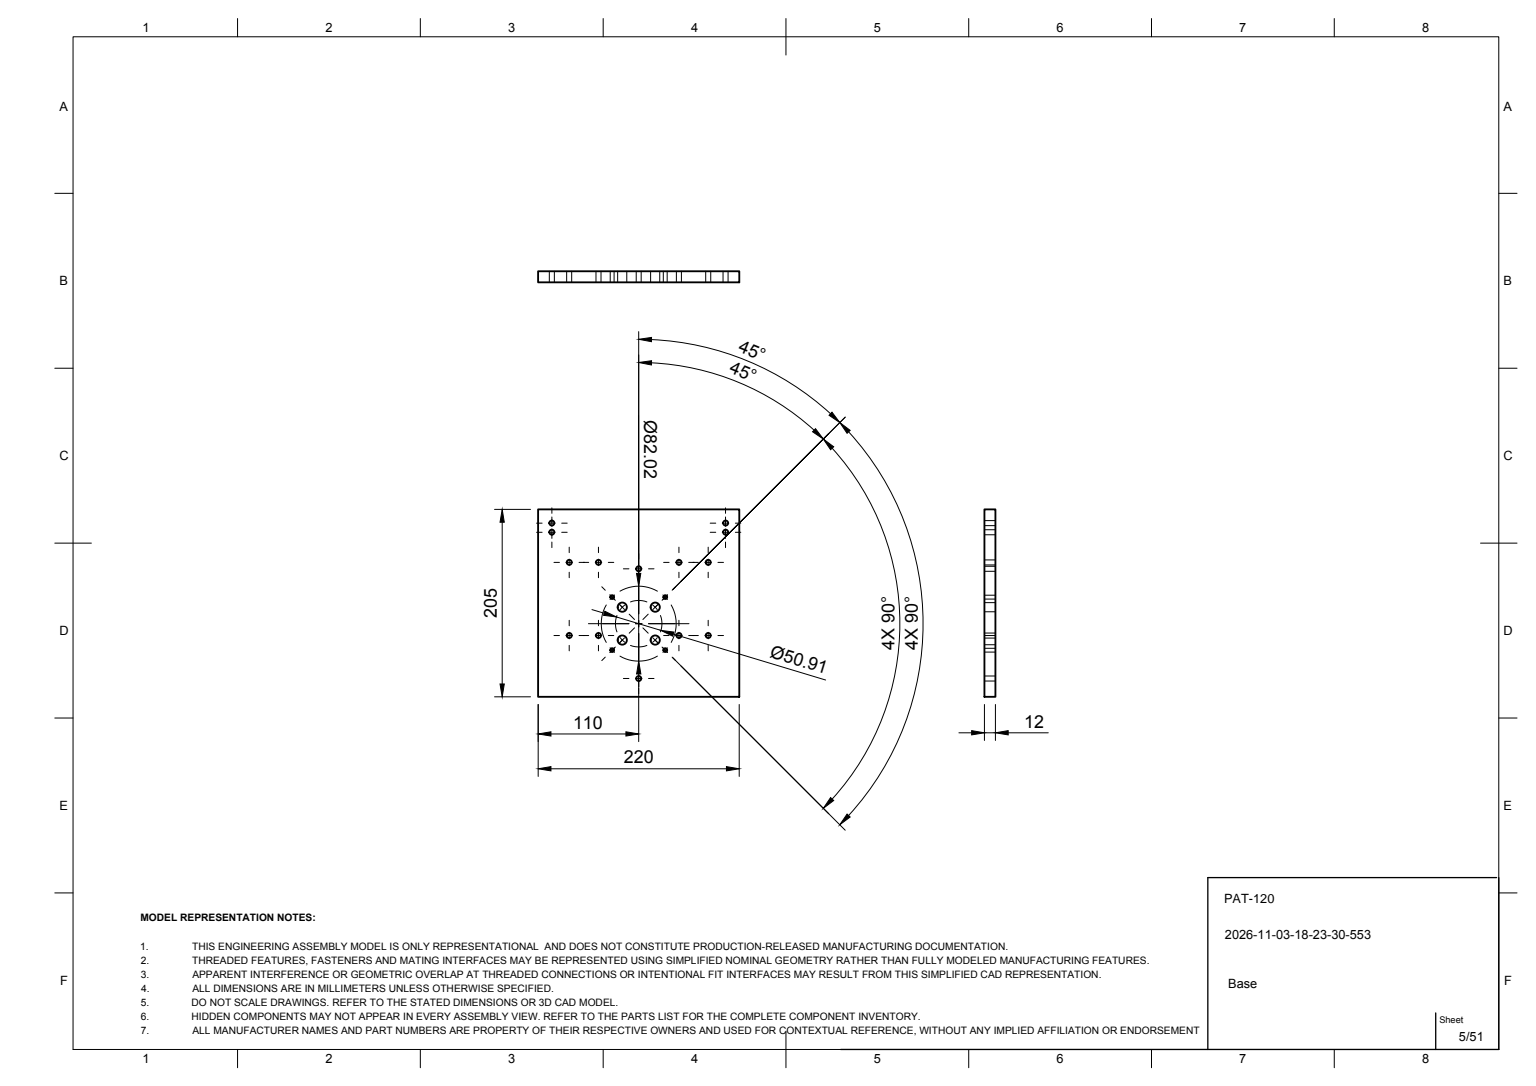
ISO-10303-21;
HEADER;
/* Generated by software containing ST-Developer
 * from STEP Tools, Inc. (www.steptools.com) 
 */

FILE_DESCRIPTION(
/* description */ ('Vibration shaker table dummy'),
/* implementation_level */ '2;1');

FILE_NAME(
/* name */ 'Base.step',
/* time_stamp */ '2026-10-27T10:55:14-07:00',
/* author */ (''),
/* organization */ (''),
/* preprocessor_version */ 'ST-DEVELOPER v20.2',
/* originating_system */ 'Autodesk Translation Framework v15.17.0.0',
/* authorisation */ '');

FILE_SCHEMA (('AUTOMOTIVE_DESIGN { 1 0 10303 214 3 1 1 }'));
ENDSEC;

DATA;
#10=MECHANICAL_DESIGN_GEOMETRIC_PRESENTATION_REPRESENTATION('',(#686),#22394);
#594=SHAPE_REPRESENTATION_RELATIONSHIP('SRR','None',#22640,#640);
#640=ADVANCED_BREP_SHAPE_REPRESENTATION('',(#732),#22346);
#686=STYLED_ITEM('',(#22940),#732);
#732=MANIFOLD_SOLID_BREP('Body1',#9204);
#775=FACE_BOUND('',#1866,.T.);
#776=FACE_BOUND('',#1867,.T.);
#777=FACE_BOUND('',#1868,.T.);
#778=FACE_BOUND('',#1869,.T.);
#779=FACE_BOUND('',#1870,.T.);
#780=FACE_BOUND('',#1871,.T.);
#781=FACE_BOUND('',#1872,.T.);
#782=FACE_BOUND('',#1873,.T.);
#783=FACE_BOUND('',#1874,.T.);
#784=FACE_BOUND('',#1875,.T.);
#785=FACE_BOUND('',#1876,.T.);
#786=FACE_BOUND('',#1877,.T.);
#787=FACE_BOUND('',#1878,.T.);
#788=FACE_BOUND('',#1879,.T.);
#789=FACE_BOUND('',#1880,.T.);
#790=FACE_BOUND('',#1881,.T.);
#791=FACE_BOUND('',#1882,.T.);
#792=FACE_BOUND('',#1883,.T.);
#793=FACE_BOUND('',#1884,.T.);
#794=FACE_BOUND('',#1885,.T.);
#795=FACE_BOUND('',#1886,.T.);
#796=FACE_BOUND('',#1887,.T.);
#797=FACE_BOUND('',#1889,.T.);
#798=FACE_BOUND('',#1890,.T.);
#799=FACE_BOUND('',#1891,.T.);
#800=FACE_BOUND('',#1892,.T.);
#801=FACE_BOUND('',#1893,.T.);
#802=FACE_BOUND('',#1894,.T.);
#803=FACE_BOUND('',#1895,.T.);
#804=FACE_BOUND('',#1896,.T.);
#805=FACE_BOUND('',#1897,.T.);
#806=FACE_BOUND('',#1898,.T.);
#807=FACE_BOUND('',#1899,.T.);
#808=FACE_BOUND('',#1900,.T.);
#809=FACE_BOUND('',#1901,.T.);
#810=FACE_BOUND('',#1902,.T.);
#811=FACE_BOUND('',#1903,.T.);
#812=FACE_BOUND('',#1904,.T.);
#813=FACE_BOUND('',#1905,.T.);
#814=FACE_BOUND('',#1906,.T.);
#815=FACE_BOUND('',#1907,.T.);
#816=FACE_BOUND('',#1908,.T.);
#817=FACE_BOUND('',#1909,.T.);
#818=FACE_BOUND('',#1910,.T.);
#1060=PLANE('',#9829);
#1061=PLANE('',#9830);
#1062=PLANE('',#9831);
#1063=PLANE('',#9832);
#1064=PLANE('',#9833);
#1065=PLANE('',#9834);
#1341=FACE_OUTER_BOUND('',#1839,.T.);
#1342=FACE_OUTER_BOUND('',#1840,.T.);
#1343=FACE_OUTER_BOUND('',#1841,.T.);
#1344=FACE_OUTER_BOUND('',#1842,.T.);
#1345=FACE_OUTER_BOUND('',#1843,.T.);
#1346=FACE_OUTER_BOUND('',#1844,.T.);
#1347=FACE_OUTER_BOUND('',#1845,.T.);
#1348=FACE_OUTER_BOUND('',#1846,.T.);
#1349=FACE_OUTER_BOUND('',#1847,.T.);
#1350=FACE_OUTER_BOUND('',#1848,.T.);
#1351=FACE_OUTER_BOUND('',#1849,.T.);
#1352=FACE_OUTER_BOUND('',#1850,.T.);
#1353=FACE_OUTER_BOUND('',#1851,.T.);
#1354=FACE_OUTER_BOUND('',#1852,.T.);
#1355=FACE_OUTER_BOUND('',#1853,.T.);
#1356=FACE_OUTER_BOUND('',#1854,.T.);
#1357=FACE_OUTER_BOUND('',#1855,.T.);
#1358=FACE_OUTER_BOUND('',#1856,.T.);
#1359=FACE_OUTER_BOUND('',#1857,.T.);
#1360=FACE_OUTER_BOUND('',#1858,.T.);
#1361=FACE_OUTER_BOUND('',#1859,.T.);
#1362=FACE_OUTER_BOUND('',#1860,.T.);
#1363=FACE_OUTER_BOUND('',#1861,.T.);
#1364=FACE_OUTER_BOUND('',#1862,.T.);
#1365=FACE_OUTER_BOUND('',#1863,.T.);
#1366=FACE_OUTER_BOUND('',#1864,.T.);
#1367=FACE_OUTER_BOUND('',#1865,.T.);
#1368=FACE_OUTER_BOUND('',#1888,.T.);
#1839=EDGE_LOOP('',(#6246,#6247,#6248,#6249));
#1840=EDGE_LOOP('',(#6250,#6251,#6252,#6253));
#1841=EDGE_LOOP('',(#6254,#6255,#6256,#6257));
#1842=EDGE_LOOP('',(#6258,#6259,#6260,#6261));
#1843=EDGE_LOOP('',(#6262,#6263,#6264,#6265));
#1844=EDGE_LOOP('',(#6266,#6267,#6268,#6269));
#1845=EDGE_LOOP('',(#6270,#6271,#6272,#6273));
#1846=EDGE_LOOP('',(#6274,#6275,#6276,#6277));
#1847=EDGE_LOOP('',(#6278,#6279,#6280,#6281));
#1848=EDGE_LOOP('',(#6282,#6283,#6284,#6285));
#1849=EDGE_LOOP('',(#6286,#6287,#6288,#6289));
#1850=EDGE_LOOP('',(#6290,#6291,#6292,#6293));
#1851=EDGE_LOOP('',(#6294,#6295,#6296,#6297));
#1852=EDGE_LOOP('',(#6298,#6299,#6300,#6301));
#1853=EDGE_LOOP('',(#6302,#6303,#6304,#6305));
#1854=EDGE_LOOP('',(#6306,#6307,#6308,#6309));
#1855=EDGE_LOOP('',(#6310,#6311,#6312,#6313));
#1856=EDGE_LOOP('',(#6314,#6315,#6316,#6317));
#1857=EDGE_LOOP('',(#6318,#6319,#6320,#6321));
#1858=EDGE_LOOP('',(#6322,#6323,#6324,#6325));
#1859=EDGE_LOOP('',(#6326,#6327,#6328,#6329));
#1860=EDGE_LOOP('',(#6330,#6331,#6332,#6333));
#1861=EDGE_LOOP('',(#6334,#6335,#6336,#6337));
#1862=EDGE_LOOP('',(#6338,#6339,#6340,#6341));
#1863=EDGE_LOOP('',(#6342,#6343,#6344,#6345));
#1864=EDGE_LOOP('',(#6346,#6347,#6348,#6349));
#1865=EDGE_LOOP('',(#6350,#6351,#6352,#6353));
#1866=EDGE_LOOP('',(#6354));
#1867=EDGE_LOOP('',(#6355));
#1868=EDGE_LOOP('',(#6356));
#1869=EDGE_LOOP('',(#6357));
#1870=EDGE_LOOP('',(#6358));
#1871=EDGE_LOOP('',(#6359));
#1872=EDGE_LOOP('',(#6360));
#1873=EDGE_LOOP('',(#6361));
#1874=EDGE_LOOP('',(#6362));
#1875=EDGE_LOOP('',(#6363));
#1876=EDGE_LOOP('',(#6364));
#1877=EDGE_LOOP('',(#6365));
#1878=EDGE_LOOP('',(#6366));
#1879=EDGE_LOOP('',(#6367));
#1880=EDGE_LOOP('',(#6368));
#1881=EDGE_LOOP('',(#6369));
#1882=EDGE_LOOP('',(#6370));
#1883=EDGE_LOOP('',(#6371));
#1884=EDGE_LOOP('',(#6372));
#1885=EDGE_LOOP('',(#6373));
#1886=EDGE_LOOP('',(#6374));
#1887=EDGE_LOOP('',(#6375));
#1888=EDGE_LOOP('',(#6376,#6377,#6378,#6379));
#1889=EDGE_LOOP('',(#6380));
#1890=EDGE_LOOP('',(#6381));
#1891=EDGE_LOOP('',(#6382));
#1892=EDGE_LOOP('',(#6383));
#1893=EDGE_LOOP('',(#6384));
#1894=EDGE_LOOP('',(#6385));
#1895=EDGE_LOOP('',(#6386));
#1896=EDGE_LOOP('',(#6387));
#1897=EDGE_LOOP('',(#6388));
#1898=EDGE_LOOP('',(#6389));
#1899=EDGE_LOOP('',(#6390));
#1900=EDGE_LOOP('',(#6391));
#1901=EDGE_LOOP('',(#6392));
#1902=EDGE_LOOP('',(#6393));
#1903=EDGE_LOOP('',(#6394));
#1904=EDGE_LOOP('',(#6395));
#1905=EDGE_LOOP('',(#6396));
#1906=EDGE_LOOP('',(#6397));
#1907=EDGE_LOOP('',(#6398));
#1908=EDGE_LOOP('',(#6399));
#1909=EDGE_LOOP('',(#6400));
#1910=EDGE_LOOP('',(#6401));
#2622=LINE('',#13956,#3241);
#2623=LINE('',#13962,#3242);
#2624=LINE('',#13968,#3243);
#2625=LINE('',#13974,#3244);
#2626=LINE('',#13980,#3245);
#2627=LINE('',#13986,#3246);
#2628=LINE('',#13992,#3247);
#2629=LINE('',#13998,#3248);
#2630=LINE('',#14004,#3249);
#2631=LINE('',#14010,#3250);
#2632=LINE('',#14016,#3251);
#2633=LINE('',#14022,#3252);
#2634=LINE('',#14028,#3253);
#2635=LINE('',#14034,#3254);
#2636=LINE('',#14040,#3255);
#2637=LINE('',#14046,#3256);
#2638=LINE('',#14052,#3257);
#2639=LINE('',#14058,#3258);
#2640=LINE('',#14064,#3259);
#2641=LINE('',#14070,#3260);
#2642=LINE('',#14076,#3261);
#2643=LINE('',#14082,#3262);
#2644=LINE('',#14087,#3263);
#2645=LINE('',#14089,#3264);
#2646=LINE('',#14091,#3265);
#2647=LINE('',#14092,#3266);
#2648=LINE('',#14095,#3267);
#2649=LINE('',#14097,#3268);
#2650=LINE('',#14098,#3269);
#2651=LINE('',#14101,#3270);
#2652=LINE('',#14103,#3271);
#2653=LINE('',#14104,#3272);
#2654=LINE('',#14106,#3273);
#2655=LINE('',#14107,#3274);
#3241=VECTOR('',#10960,0.275);
#3242=VECTOR('',#10967,0.275);
#3243=VECTOR('',#10974,0.5);
#3244=VECTOR('',#10981,0.5);
#3245=VECTOR('',#10988,0.5);
#3246=VECTOR('',#10995,0.5);
#3247=VECTOR('',#11002,0.21);
#3248=VECTOR('',#11009,0.21);
#3249=VECTOR('',#11016,0.21);
#3250=VECTOR('',#11023,0.21);
#3251=VECTOR('',#11030,0.275);
#3252=VECTOR('',#11037,0.275);
#3253=VECTOR('',#11044,0.275);
#3254=VECTOR('',#11051,0.275);
#3255=VECTOR('',#11058,0.275);
#3256=VECTOR('',#11065,0.275);
#3257=VECTOR('',#11072,0.275);
#3258=VECTOR('',#11079,0.275);
#3259=VECTOR('',#11086,0.275);
#3260=VECTOR('',#11093,0.275);
#3261=VECTOR('',#11100,0.275);
#3262=VECTOR('',#11107,0.275);
#3263=VECTOR('',#11112,1.);
#3264=VECTOR('',#11113,1.);
#3265=VECTOR('',#11114,1.);
#3266=VECTOR('',#11115,1.);
#3267=VECTOR('',#11118,1.);
#3268=VECTOR('',#11119,1.);
#3269=VECTOR('',#11120,1.);
#3270=VECTOR('',#11123,1.);
#3271=VECTOR('',#11124,1.);
#3272=VECTOR('',#11125,1.);
#3273=VECTOR('',#11128,1.);
#3274=VECTOR('',#11129,1.);
#3860=CIRCLE('',#9764,0.275);
#3861=CIRCLE('',#9765,0.275);
#3862=CIRCLE('',#9767,0.275);
#3863=CIRCLE('',#9768,0.275);
#3864=CIRCLE('',#9770,0.5);
#3865=CIRCLE('',#9771,0.5);
#3866=CIRCLE('',#9773,0.5);
#3867=CIRCLE('',#9774,0.5);
#3868=CIRCLE('',#9776,0.5);
#3869=CIRCLE('',#9777,0.5);
#3870=CIRCLE('',#9779,0.5);
#3871=CIRCLE('',#9780,0.5);
#3872=CIRCLE('',#9782,0.21);
#3873=CIRCLE('',#9783,0.21);
#3874=CIRCLE('',#9785,0.21);
#3875=CIRCLE('',#9786,0.21);
#3876=CIRCLE('',#9788,0.21);
#3877=CIRCLE('',#9789,0.21);
#3878=CIRCLE('',#9791,0.21);
#3879=CIRCLE('',#9792,0.21);
#3880=CIRCLE('',#9794,0.275);
#3881=CIRCLE('',#9795,0.275);
#3882=CIRCLE('',#9797,0.275);
#3883=CIRCLE('',#9798,0.275);
#3884=CIRCLE('',#9800,0.275);
#3885=CIRCLE('',#9801,0.275);
#3886=CIRCLE('',#9803,0.275);
#3887=CIRCLE('',#9804,0.275);
#3888=CIRCLE('',#9806,0.275);
#3889=CIRCLE('',#9807,0.275);
#3890=CIRCLE('',#9809,0.275);
#3891=CIRCLE('',#9810,0.275);
#3892=CIRCLE('',#9812,0.275);
#3893=CIRCLE('',#9813,0.275);
#3894=CIRCLE('',#9815,0.275);
#3895=CIRCLE('',#9816,0.275);
#3896=CIRCLE('',#9818,0.275);
#3897=CIRCLE('',#9819,0.275);
#3898=CIRCLE('',#9821,0.275);
#3899=CIRCLE('',#9822,0.275);
#3900=CIRCLE('',#9824,0.275);
#3901=CIRCLE('',#9825,0.275);
#3902=CIRCLE('',#9827,0.275);
#3903=CIRCLE('',#9828,0.275);
#4367=VERTEX_POINT('',#13953);
#4368=VERTEX_POINT('',#13955);
#4369=VERTEX_POINT('',#13959);
#4370=VERTEX_POINT('',#13961);
#4371=VERTEX_POINT('',#13965);
#4372=VERTEX_POINT('',#13967);
#4373=VERTEX_POINT('',#13971);
#4374=VERTEX_POINT('',#13973);
#4375=VERTEX_POINT('',#13977);
#4376=VERTEX_POINT('',#13979);
#4377=VERTEX_POINT('',#13983);
#4378=VERTEX_POINT('',#13985);
#4379=VERTEX_POINT('',#13989);
#4380=VERTEX_POINT('',#13991);
#4381=VERTEX_POINT('',#13995);
#4382=VERTEX_POINT('',#13997);
#4383=VERTEX_POINT('',#14001);
#4384=VERTEX_POINT('',#14003);
#4385=VERTEX_POINT('',#14007);
#4386=VERTEX_POINT('',#14009);
#4387=VERTEX_POINT('',#14013);
#4388=VERTEX_POINT('',#14015);
#4389=VERTEX_POINT('',#14019);
#4390=VERTEX_POINT('',#14021);
#4391=VERTEX_POINT('',#14025);
#4392=VERTEX_POINT('',#14027);
#4393=VERTEX_POINT('',#14031);
#4394=VERTEX_POINT('',#14033);
#4395=VERTEX_POINT('',#14037);
#4396=VERTEX_POINT('',#14039);
#4397=VERTEX_POINT('',#14043);
#4398=VERTEX_POINT('',#14045);
#4399=VERTEX_POINT('',#14049);
#4400=VERTEX_POINT('',#14051);
#4401=VERTEX_POINT('',#14055);
#4402=VERTEX_POINT('',#14057);
#4403=VERTEX_POINT('',#14061);
#4404=VERTEX_POINT('',#14063);
#4405=VERTEX_POINT('',#14067);
#4406=VERTEX_POINT('',#14069);
#4407=VERTEX_POINT('',#14073);
#4408=VERTEX_POINT('',#14075);
#4409=VERTEX_POINT('',#14079);
#4410=VERTEX_POINT('',#14081);
#4411=VERTEX_POINT('',#14085);
#4412=VERTEX_POINT('',#14086);
#4413=VERTEX_POINT('',#14088);
#4414=VERTEX_POINT('',#14090);
#4415=VERTEX_POINT('',#14094);
#4416=VERTEX_POINT('',#14096);
#4417=VERTEX_POINT('',#14100);
#4418=VERTEX_POINT('',#14102);
#5116=EDGE_CURVE('',#4367,#4367,#3860,.T.);
#5117=EDGE_CURVE('',#4367,#4368,#2622,.T.);
#5118=EDGE_CURVE('',#4368,#4368,#3861,.T.);
#5119=EDGE_CURVE('',#4369,#4369,#3862,.T.);
#5120=EDGE_CURVE('',#4369,#4370,#2623,.T.);
#5121=EDGE_CURVE('',#4370,#4370,#3863,.T.);
#5122=EDGE_CURVE('',#4371,#4371,#3864,.T.);
#5123=EDGE_CURVE('',#4371,#4372,#2624,.T.);
#5124=EDGE_CURVE('',#4372,#4372,#3865,.T.);
#5125=EDGE_CURVE('',#4373,#4373,#3866,.T.);
#5126=EDGE_CURVE('',#4373,#4374,#2625,.T.);
#5127=EDGE_CURVE('',#4374,#4374,#3867,.T.);
#5128=EDGE_CURVE('',#4375,#4375,#3868,.T.);
#5129=EDGE_CURVE('',#4375,#4376,#2626,.T.);
#5130=EDGE_CURVE('',#4376,#4376,#3869,.T.);
#5131=EDGE_CURVE('',#4377,#4377,#3870,.T.);
#5132=EDGE_CURVE('',#4377,#4378,#2627,.T.);
#5133=EDGE_CURVE('',#4378,#4378,#3871,.T.);
#5134=EDGE_CURVE('',#4379,#4379,#3872,.T.);
#5135=EDGE_CURVE('',#4379,#4380,#2628,.T.);
#5136=EDGE_CURVE('',#4380,#4380,#3873,.T.);
#5137=EDGE_CURVE('',#4381,#4381,#3874,.T.);
#5138=EDGE_CURVE('',#4381,#4382,#2629,.T.);
#5139=EDGE_CURVE('',#4382,#4382,#3875,.T.);
#5140=EDGE_CURVE('',#4383,#4383,#3876,.T.);
#5141=EDGE_CURVE('',#4383,#4384,#2630,.T.);
#5142=EDGE_CURVE('',#4384,#4384,#3877,.T.);
#5143=EDGE_CURVE('',#4385,#4385,#3878,.T.);
#5144=EDGE_CURVE('',#4385,#4386,#2631,.T.);
#5145=EDGE_CURVE('',#4386,#4386,#3879,.T.);
#5146=EDGE_CURVE('',#4387,#4387,#3880,.T.);
#5147=EDGE_CURVE('',#4387,#4388,#2632,.T.);
#5148=EDGE_CURVE('',#4388,#4388,#3881,.T.);
#5149=EDGE_CURVE('',#4389,#4389,#3882,.T.);
#5150=EDGE_CURVE('',#4389,#4390,#2633,.T.);
#5151=EDGE_CURVE('',#4390,#4390,#3883,.T.);
#5152=EDGE_CURVE('',#4391,#4391,#3884,.T.);
#5153=EDGE_CURVE('',#4391,#4392,#2634,.T.);
#5154=EDGE_CURVE('',#4392,#4392,#3885,.T.);
#5155=EDGE_CURVE('',#4393,#4393,#3886,.T.);
#5156=EDGE_CURVE('',#4393,#4394,#2635,.T.);
#5157=EDGE_CURVE('',#4394,#4394,#3887,.T.);
#5158=EDGE_CURVE('',#4395,#4395,#3888,.T.);
#5159=EDGE_CURVE('',#4395,#4396,#2636,.T.);
#5160=EDGE_CURVE('',#4396,#4396,#3889,.T.);
#5161=EDGE_CURVE('',#4397,#4397,#3890,.T.);
#5162=EDGE_CURVE('',#4397,#4398,#2637,.T.);
#5163=EDGE_CURVE('',#4398,#4398,#3891,.T.);
#5164=EDGE_CURVE('',#4399,#4399,#3892,.T.);
#5165=EDGE_CURVE('',#4399,#4400,#2638,.T.);
#5166=EDGE_CURVE('',#4400,#4400,#3893,.T.);
#5167=EDGE_CURVE('',#4401,#4401,#3894,.T.);
#5168=EDGE_CURVE('',#4401,#4402,#2639,.T.);
#5169=EDGE_CURVE('',#4402,#4402,#3895,.T.);
#5170=EDGE_CURVE('',#4403,#4403,#3896,.T.);
#5171=EDGE_CURVE('',#4403,#4404,#2640,.T.);
#5172=EDGE_CURVE('',#4404,#4404,#3897,.T.);
#5173=EDGE_CURVE('',#4405,#4405,#3898,.T.);
#5174=EDGE_CURVE('',#4405,#4406,#2641,.T.);
#5175=EDGE_CURVE('',#4406,#4406,#3899,.T.);
#5176=EDGE_CURVE('',#4407,#4407,#3900,.T.);
#5177=EDGE_CURVE('',#4407,#4408,#2642,.T.);
#5178=EDGE_CURVE('',#4408,#4408,#3901,.T.);
#5179=EDGE_CURVE('',#4409,#4409,#3902,.T.);
#5180=EDGE_CURVE('',#4409,#4410,#2643,.T.);
#5181=EDGE_CURVE('',#4410,#4410,#3903,.T.);
#5182=EDGE_CURVE('',#4411,#4412,#2644,.T.);
#5183=EDGE_CURVE('',#4412,#4413,#2645,.T.);
#5184=EDGE_CURVE('',#4414,#4413,#2646,.T.);
#5185=EDGE_CURVE('',#4411,#4414,#2647,.T.);
#5186=EDGE_CURVE('',#4415,#4411,#2648,.T.);
#5187=EDGE_CURVE('',#4416,#4414,#2649,.T.);
#5188=EDGE_CURVE('',#4415,#4416,#2650,.T.);
#5189=EDGE_CURVE('',#4417,#4415,#2651,.T.);
#5190=EDGE_CURVE('',#4418,#4416,#2652,.T.);
#5191=EDGE_CURVE('',#4417,#4418,#2653,.T.);
#5192=EDGE_CURVE('',#4412,#4417,#2654,.T.);
#5193=EDGE_CURVE('',#4413,#4418,#2655,.T.);
#6246=ORIENTED_EDGE('',*,*,#5116,.F.);
#6247=ORIENTED_EDGE('',*,*,#5117,.T.);
#6248=ORIENTED_EDGE('',*,*,#5118,.F.);
#6249=ORIENTED_EDGE('',*,*,#5117,.F.);
#6250=ORIENTED_EDGE('',*,*,#5119,.F.);
#6251=ORIENTED_EDGE('',*,*,#5120,.T.);
#6252=ORIENTED_EDGE('',*,*,#5121,.F.);
#6253=ORIENTED_EDGE('',*,*,#5120,.F.);
#6254=ORIENTED_EDGE('',*,*,#5122,.F.);
#6255=ORIENTED_EDGE('',*,*,#5123,.T.);
#6256=ORIENTED_EDGE('',*,*,#5124,.F.);
#6257=ORIENTED_EDGE('',*,*,#5123,.F.);
#6258=ORIENTED_EDGE('',*,*,#5125,.F.);
#6259=ORIENTED_EDGE('',*,*,#5126,.T.);
#6260=ORIENTED_EDGE('',*,*,#5127,.F.);
#6261=ORIENTED_EDGE('',*,*,#5126,.F.);
#6262=ORIENTED_EDGE('',*,*,#5128,.F.);
#6263=ORIENTED_EDGE('',*,*,#5129,.T.);
#6264=ORIENTED_EDGE('',*,*,#5130,.F.);
#6265=ORIENTED_EDGE('',*,*,#5129,.F.);
#6266=ORIENTED_EDGE('',*,*,#5131,.F.);
#6267=ORIENTED_EDGE('',*,*,#5132,.T.);
#6268=ORIENTED_EDGE('',*,*,#5133,.F.);
#6269=ORIENTED_EDGE('',*,*,#5132,.F.);
#6270=ORIENTED_EDGE('',*,*,#5134,.F.);
#6271=ORIENTED_EDGE('',*,*,#5135,.T.);
#6272=ORIENTED_EDGE('',*,*,#5136,.F.);
#6273=ORIENTED_EDGE('',*,*,#5135,.F.);
#6274=ORIENTED_EDGE('',*,*,#5137,.F.);
#6275=ORIENTED_EDGE('',*,*,#5138,.T.);
#6276=ORIENTED_EDGE('',*,*,#5139,.F.);
#6277=ORIENTED_EDGE('',*,*,#5138,.F.);
#6278=ORIENTED_EDGE('',*,*,#5140,.F.);
#6279=ORIENTED_EDGE('',*,*,#5141,.T.);
#6280=ORIENTED_EDGE('',*,*,#5142,.F.);
#6281=ORIENTED_EDGE('',*,*,#5141,.F.);
#6282=ORIENTED_EDGE('',*,*,#5143,.F.);
#6283=ORIENTED_EDGE('',*,*,#5144,.T.);
#6284=ORIENTED_EDGE('',*,*,#5145,.F.);
#6285=ORIENTED_EDGE('',*,*,#5144,.F.);
#6286=ORIENTED_EDGE('',*,*,#5146,.F.);
#6287=ORIENTED_EDGE('',*,*,#5147,.T.);
#6288=ORIENTED_EDGE('',*,*,#5148,.F.);
#6289=ORIENTED_EDGE('',*,*,#5147,.F.);
#6290=ORIENTED_EDGE('',*,*,#5149,.F.);
#6291=ORIENTED_EDGE('',*,*,#5150,.T.);
#6292=ORIENTED_EDGE('',*,*,#5151,.F.);
#6293=ORIENTED_EDGE('',*,*,#5150,.F.);
#6294=ORIENTED_EDGE('',*,*,#5152,.F.);
#6295=ORIENTED_EDGE('',*,*,#5153,.T.);
#6296=ORIENTED_EDGE('',*,*,#5154,.F.);
#6297=ORIENTED_EDGE('',*,*,#5153,.F.);
#6298=ORIENTED_EDGE('',*,*,#5155,.F.);
#6299=ORIENTED_EDGE('',*,*,#5156,.T.);
#6300=ORIENTED_EDGE('',*,*,#5157,.F.);
#6301=ORIENTED_EDGE('',*,*,#5156,.F.);
#6302=ORIENTED_EDGE('',*,*,#5158,.F.);
#6303=ORIENTED_EDGE('',*,*,#5159,.T.);
#6304=ORIENTED_EDGE('',*,*,#5160,.F.);
#6305=ORIENTED_EDGE('',*,*,#5159,.F.);
#6306=ORIENTED_EDGE('',*,*,#5161,.F.);
#6307=ORIENTED_EDGE('',*,*,#5162,.T.);
#6308=ORIENTED_EDGE('',*,*,#5163,.F.);
#6309=ORIENTED_EDGE('',*,*,#5162,.F.);
#6310=ORIENTED_EDGE('',*,*,#5164,.F.);
#6311=ORIENTED_EDGE('',*,*,#5165,.T.);
#6312=ORIENTED_EDGE('',*,*,#5166,.F.);
#6313=ORIENTED_EDGE('',*,*,#5165,.F.);
#6314=ORIENTED_EDGE('',*,*,#5167,.F.);
#6315=ORIENTED_EDGE('',*,*,#5168,.T.);
#6316=ORIENTED_EDGE('',*,*,#5169,.F.);
#6317=ORIENTED_EDGE('',*,*,#5168,.F.);
#6318=ORIENTED_EDGE('',*,*,#5170,.F.);
#6319=ORIENTED_EDGE('',*,*,#5171,.T.);
#6320=ORIENTED_EDGE('',*,*,#5172,.F.);
#6321=ORIENTED_EDGE('',*,*,#5171,.F.);
#6322=ORIENTED_EDGE('',*,*,#5173,.F.);
#6323=ORIENTED_EDGE('',*,*,#5174,.T.);
#6324=ORIENTED_EDGE('',*,*,#5175,.F.);
#6325=ORIENTED_EDGE('',*,*,#5174,.F.);
#6326=ORIENTED_EDGE('',*,*,#5176,.F.);
#6327=ORIENTED_EDGE('',*,*,#5177,.T.);
#6328=ORIENTED_EDGE('',*,*,#5178,.F.);
#6329=ORIENTED_EDGE('',*,*,#5177,.F.);
#6330=ORIENTED_EDGE('',*,*,#5179,.F.);
#6331=ORIENTED_EDGE('',*,*,#5180,.T.);
#6332=ORIENTED_EDGE('',*,*,#5181,.F.);
#6333=ORIENTED_EDGE('',*,*,#5180,.F.);
#6334=ORIENTED_EDGE('',*,*,#5182,.T.);
#6335=ORIENTED_EDGE('',*,*,#5183,.T.);
#6336=ORIENTED_EDGE('',*,*,#5184,.F.);
#6337=ORIENTED_EDGE('',*,*,#5185,.F.);
#6338=ORIENTED_EDGE('',*,*,#5186,.T.);
#6339=ORIENTED_EDGE('',*,*,#5185,.T.);
#6340=ORIENTED_EDGE('',*,*,#5187,.F.);
#6341=ORIENTED_EDGE('',*,*,#5188,.F.);
#6342=ORIENTED_EDGE('',*,*,#5189,.T.);
#6343=ORIENTED_EDGE('',*,*,#5188,.T.);
#6344=ORIENTED_EDGE('',*,*,#5190,.F.);
#6345=ORIENTED_EDGE('',*,*,#5191,.F.);
#6346=ORIENTED_EDGE('',*,*,#5192,.T.);
#6347=ORIENTED_EDGE('',*,*,#5191,.T.);
#6348=ORIENTED_EDGE('',*,*,#5193,.F.);
#6349=ORIENTED_EDGE('',*,*,#5183,.F.);
#6350=ORIENTED_EDGE('',*,*,#5193,.T.);
#6351=ORIENTED_EDGE('',*,*,#5190,.T.);
#6352=ORIENTED_EDGE('',*,*,#5187,.T.);
#6353=ORIENTED_EDGE('',*,*,#5184,.T.);
#6354=ORIENTED_EDGE('',*,*,#5121,.T.);
#6355=ORIENTED_EDGE('',*,*,#5136,.T.);
#6356=ORIENTED_EDGE('',*,*,#5139,.T.);
#6357=ORIENTED_EDGE('',*,*,#5142,.T.);
#6358=ORIENTED_EDGE('',*,*,#5145,.T.);
#6359=ORIENTED_EDGE('',*,*,#5154,.T.);
#6360=ORIENTED_EDGE('',*,*,#5157,.T.);
#6361=ORIENTED_EDGE('',*,*,#5181,.T.);
#6362=ORIENTED_EDGE('',*,*,#5178,.T.);
#6363=ORIENTED_EDGE('',*,*,#5175,.T.);
#6364=ORIENTED_EDGE('',*,*,#5172,.T.);
#6365=ORIENTED_EDGE('',*,*,#5169,.T.);
#6366=ORIENTED_EDGE('',*,*,#5166,.T.);
#6367=ORIENTED_EDGE('',*,*,#5163,.T.);
#6368=ORIENTED_EDGE('',*,*,#5160,.T.);
#6369=ORIENTED_EDGE('',*,*,#5151,.T.);
#6370=ORIENTED_EDGE('',*,*,#5148,.T.);
#6371=ORIENTED_EDGE('',*,*,#5133,.T.);
#6372=ORIENTED_EDGE('',*,*,#5130,.T.);
#6373=ORIENTED_EDGE('',*,*,#5127,.T.);
#6374=ORIENTED_EDGE('',*,*,#5124,.T.);
#6375=ORIENTED_EDGE('',*,*,#5118,.T.);
#6376=ORIENTED_EDGE('',*,*,#5192,.F.);
#6377=ORIENTED_EDGE('',*,*,#5182,.F.);
#6378=ORIENTED_EDGE('',*,*,#5186,.F.);
#6379=ORIENTED_EDGE('',*,*,#5189,.F.);
#6380=ORIENTED_EDGE('',*,*,#5119,.T.);
#6381=ORIENTED_EDGE('',*,*,#5134,.T.);
#6382=ORIENTED_EDGE('',*,*,#5137,.T.);
#6383=ORIENTED_EDGE('',*,*,#5140,.T.);
#6384=ORIENTED_EDGE('',*,*,#5143,.T.);
#6385=ORIENTED_EDGE('',*,*,#5152,.T.);
#6386=ORIENTED_EDGE('',*,*,#5155,.T.);
#6387=ORIENTED_EDGE('',*,*,#5179,.T.);
#6388=ORIENTED_EDGE('',*,*,#5176,.T.);
#6389=ORIENTED_EDGE('',*,*,#5173,.T.);
#6390=ORIENTED_EDGE('',*,*,#5170,.T.);
#6391=ORIENTED_EDGE('',*,*,#5167,.T.);
#6392=ORIENTED_EDGE('',*,*,#5164,.T.);
#6393=ORIENTED_EDGE('',*,*,#5161,.T.);
#6394=ORIENTED_EDGE('',*,*,#5158,.T.);
#6395=ORIENTED_EDGE('',*,*,#5149,.T.);
#6396=ORIENTED_EDGE('',*,*,#5146,.T.);
#6397=ORIENTED_EDGE('',*,*,#5131,.T.);
#6398=ORIENTED_EDGE('',*,*,#5128,.T.);
#6399=ORIENTED_EDGE('',*,*,#5125,.T.);
#6400=ORIENTED_EDGE('',*,*,#5122,.T.);
#6401=ORIENTED_EDGE('',*,*,#5116,.T.);
#8506=CYLINDRICAL_SURFACE('',#9763,0.275);
#8507=CYLINDRICAL_SURFACE('',#9766,0.275);
#8508=CYLINDRICAL_SURFACE('',#9769,0.5);
#8509=CYLINDRICAL_SURFACE('',#9772,0.5);
#8510=CYLINDRICAL_SURFACE('',#9775,0.5);
#8511=CYLINDRICAL_SURFACE('',#9778,0.5);
#8512=CYLINDRICAL_SURFACE('',#9781,0.21);
#8513=CYLINDRICAL_SURFACE('',#9784,0.21);
#8514=CYLINDRICAL_SURFACE('',#9787,0.21);
#8515=CYLINDRICAL_SURFACE('',#9790,0.21);
#8516=CYLINDRICAL_SURFACE('',#9793,0.275);
#8517=CYLINDRICAL_SURFACE('',#9796,0.275);
#8518=CYLINDRICAL_SURFACE('',#9799,0.275);
#8519=CYLINDRICAL_SURFACE('',#9802,0.275);
#8520=CYLINDRICAL_SURFACE('',#9805,0.275);
#8521=CYLINDRICAL_SURFACE('',#9808,0.275);
#8522=CYLINDRICAL_SURFACE('',#9811,0.275);
#8523=CYLINDRICAL_SURFACE('',#9814,0.275);
#8524=CYLINDRICAL_SURFACE('',#9817,0.275);
#8525=CYLINDRICAL_SURFACE('',#9820,0.275);
#8526=CYLINDRICAL_SURFACE('',#9823,0.275);
#8527=CYLINDRICAL_SURFACE('',#9826,0.275);
#8706=ADVANCED_FACE('',(#1341),#8506,.F.);
#8707=ADVANCED_FACE('',(#1342),#8507,.F.);
#8708=ADVANCED_FACE('',(#1343),#8508,.F.);
#8709=ADVANCED_FACE('',(#1344),#8509,.F.);
#8710=ADVANCED_FACE('',(#1345),#8510,.F.);
#8711=ADVANCED_FACE('',(#1346),#8511,.F.);
#8712=ADVANCED_FACE('',(#1347),#8512,.F.);
#8713=ADVANCED_FACE('',(#1348),#8513,.F.);
#8714=ADVANCED_FACE('',(#1349),#8514,.F.);
#8715=ADVANCED_FACE('',(#1350),#8515,.F.);
#8716=ADVANCED_FACE('',(#1351),#8516,.F.);
#8717=ADVANCED_FACE('',(#1352),#8517,.F.);
#8718=ADVANCED_FACE('',(#1353),#8518,.F.);
#8719=ADVANCED_FACE('',(#1354),#8519,.F.);
#8720=ADVANCED_FACE('',(#1355),#8520,.F.);
#8721=ADVANCED_FACE('',(#1356),#8521,.F.);
#8722=ADVANCED_FACE('',(#1357),#8522,.F.);
#8723=ADVANCED_FACE('',(#1358),#8523,.F.);
#8724=ADVANCED_FACE('',(#1359),#8524,.F.);
#8725=ADVANCED_FACE('',(#1360),#8525,.F.);
#8726=ADVANCED_FACE('',(#1361),#8526,.F.);
#8727=ADVANCED_FACE('',(#1362),#8527,.F.);
#8728=ADVANCED_FACE('',(#1363),#1060,.T.);
#8729=ADVANCED_FACE('',(#1364),#1061,.T.);
#8730=ADVANCED_FACE('',(#1365),#1062,.T.);
#8731=ADVANCED_FACE('',(#1366),#1063,.T.);
#8732=ADVANCED_FACE('',(#1367,#775,#776,#777,#778,#779,#780,#781,#782,#783,
#784,#785,#786,#787,#788,#789,#790,#791,#792,#793,#794,#795,#796),#1064,
 .T.);
#8733=ADVANCED_FACE('',(#1368,#797,#798,#799,#800,#801,#802,#803,#804,#805,
#806,#807,#808,#809,#810,#811,#812,#813,#814,#815,#816,#817,#818),#1065,
 .F.);
#9204=CLOSED_SHELL('',(#8706,#8707,#8708,#8709,#8710,#8711,#8712,#8713,
#8714,#8715,#8716,#8717,#8718,#8719,#8720,#8721,#8722,#8723,#8724,#8725,
#8726,#8727,#8728,#8729,#8730,#8731,#8732,#8733));
#9762=AXIS2_PLACEMENT_3D('',#13951,#10954,#10955);
#9763=AXIS2_PLACEMENT_3D('',#13952,#10956,#10957);
#9764=AXIS2_PLACEMENT_3D('',#13954,#10958,#10959);
#9765=AXIS2_PLACEMENT_3D('',#13957,#10961,#10962);
#9766=AXIS2_PLACEMENT_3D('',#13958,#10963,#10964);
#9767=AXIS2_PLACEMENT_3D('',#13960,#10965,#10966);
#9768=AXIS2_PLACEMENT_3D('',#13963,#10968,#10969);
#9769=AXIS2_PLACEMENT_3D('',#13964,#10970,#10971);
#9770=AXIS2_PLACEMENT_3D('',#13966,#10972,#10973);
#9771=AXIS2_PLACEMENT_3D('',#13969,#10975,#10976);
#9772=AXIS2_PLACEMENT_3D('',#13970,#10977,#10978);
#9773=AXIS2_PLACEMENT_3D('',#13972,#10979,#10980);
#9774=AXIS2_PLACEMENT_3D('',#13975,#10982,#10983);
#9775=AXIS2_PLACEMENT_3D('',#13976,#10984,#10985);
#9776=AXIS2_PLACEMENT_3D('',#13978,#10986,#10987);
#9777=AXIS2_PLACEMENT_3D('',#13981,#10989,#10990);
#9778=AXIS2_PLACEMENT_3D('',#13982,#10991,#10992);
#9779=AXIS2_PLACEMENT_3D('',#13984,#10993,#10994);
#9780=AXIS2_PLACEMENT_3D('',#13987,#10996,#10997);
#9781=AXIS2_PLACEMENT_3D('',#13988,#10998,#10999);
#9782=AXIS2_PLACEMENT_3D('',#13990,#11000,#11001);
#9783=AXIS2_PLACEMENT_3D('',#13993,#11003,#11004);
#9784=AXIS2_PLACEMENT_3D('',#13994,#11005,#11006);
#9785=AXIS2_PLACEMENT_3D('',#13996,#11007,#11008);
#9786=AXIS2_PLACEMENT_3D('',#13999,#11010,#11011);
#9787=AXIS2_PLACEMENT_3D('',#14000,#11012,#11013);
#9788=AXIS2_PLACEMENT_3D('',#14002,#11014,#11015);
#9789=AXIS2_PLACEMENT_3D('',#14005,#11017,#11018);
#9790=AXIS2_PLACEMENT_3D('',#14006,#11019,#11020);
#9791=AXIS2_PLACEMENT_3D('',#14008,#11021,#11022);
#9792=AXIS2_PLACEMENT_3D('',#14011,#11024,#11025);
#9793=AXIS2_PLACEMENT_3D('',#14012,#11026,#11027);
#9794=AXIS2_PLACEMENT_3D('',#14014,#11028,#11029);
#9795=AXIS2_PLACEMENT_3D('',#14017,#11031,#11032);
#9796=AXIS2_PLACEMENT_3D('',#14018,#11033,#11034);
#9797=AXIS2_PLACEMENT_3D('',#14020,#11035,#11036);
#9798=AXIS2_PLACEMENT_3D('',#14023,#11038,#11039);
#9799=AXIS2_PLACEMENT_3D('',#14024,#11040,#11041);
#9800=AXIS2_PLACEMENT_3D('',#14026,#11042,#11043);
#9801=AXIS2_PLACEMENT_3D('',#14029,#11045,#11046);
#9802=AXIS2_PLACEMENT_3D('',#14030,#11047,#11048);
#9803=AXIS2_PLACEMENT_3D('',#14032,#11049,#11050);
#9804=AXIS2_PLACEMENT_3D('',#14035,#11052,#11053);
#9805=AXIS2_PLACEMENT_3D('',#14036,#11054,#11055);
#9806=AXIS2_PLACEMENT_3D('',#14038,#11056,#11057);
#9807=AXIS2_PLACEMENT_3D('',#14041,#11059,#11060);
#9808=AXIS2_PLACEMENT_3D('',#14042,#11061,#11062);
#9809=AXIS2_PLACEMENT_3D('',#14044,#11063,#11064);
#9810=AXIS2_PLACEMENT_3D('',#14047,#11066,#11067);
#9811=AXIS2_PLACEMENT_3D('',#14048,#11068,#11069);
#9812=AXIS2_PLACEMENT_3D('',#14050,#11070,#11071);
#9813=AXIS2_PLACEMENT_3D('',#14053,#11073,#11074);
#9814=AXIS2_PLACEMENT_3D('',#14054,#11075,#11076);
#9815=AXIS2_PLACEMENT_3D('',#14056,#11077,#11078);
#9816=AXIS2_PLACEMENT_3D('',#14059,#11080,#11081);
#9817=AXIS2_PLACEMENT_3D('',#14060,#11082,#11083);
#9818=AXIS2_PLACEMENT_3D('',#14062,#11084,#11085);
#9819=AXIS2_PLACEMENT_3D('',#14065,#11087,#11088);
#9820=AXIS2_PLACEMENT_3D('',#14066,#11089,#11090);
#9821=AXIS2_PLACEMENT_3D('',#14068,#11091,#11092);
#9822=AXIS2_PLACEMENT_3D('',#14071,#11094,#11095);
#9823=AXIS2_PLACEMENT_3D('',#14072,#11096,#11097);
#9824=AXIS2_PLACEMENT_3D('',#14074,#11098,#11099);
#9825=AXIS2_PLACEMENT_3D('',#14077,#11101,#11102);
#9826=AXIS2_PLACEMENT_3D('',#14078,#11103,#11104);
#9827=AXIS2_PLACEMENT_3D('',#14080,#11105,#11106);
#9828=AXIS2_PLACEMENT_3D('',#14083,#11108,#11109);
#9829=AXIS2_PLACEMENT_3D('',#14084,#11110,#11111);
#9830=AXIS2_PLACEMENT_3D('',#14093,#11116,#11117);
#9831=AXIS2_PLACEMENT_3D('',#14099,#11121,#11122);
#9832=AXIS2_PLACEMENT_3D('',#14105,#11126,#11127);
#9833=AXIS2_PLACEMENT_3D('',#14108,#11130,#11131);
#9834=AXIS2_PLACEMENT_3D('',#14109,#11132,#11133);
#10954=DIRECTION('axis',(0.,0.,1.));
#10955=DIRECTION('refdir',(1.,0.,0.));
#10956=DIRECTION('center_axis',(0.,0.,1.));
#10957=DIRECTION('ref_axis',(1.,0.,0.));
#10958=DIRECTION('center_axis',(0.,0.,1.));
#10959=DIRECTION('ref_axis',(1.,0.,0.));
#10960=DIRECTION('',(0.,0.,1.));
#10961=DIRECTION('center_axis',(0.,0.,-1.));
#10962=DIRECTION('ref_axis',(1.,0.,0.));
#10963=DIRECTION('center_axis',(0.,0.,1.));
#10964=DIRECTION('ref_axis',(1.,0.,0.));
#10965=DIRECTION('center_axis',(0.,0.,1.));
#10966=DIRECTION('ref_axis',(1.,0.,0.));
#10967=DIRECTION('',(0.,0.,1.));
#10968=DIRECTION('center_axis',(0.,0.,-1.));
#10969=DIRECTION('ref_axis',(1.,0.,0.));
#10970=DIRECTION('center_axis',(0.,0.,1.));
#10971=DIRECTION('ref_axis',(1.,0.,0.));
#10972=DIRECTION('center_axis',(0.,0.,1.));
#10973=DIRECTION('ref_axis',(1.,0.,0.));
#10974=DIRECTION('',(0.,0.,1.));
#10975=DIRECTION('center_axis',(0.,0.,-1.));
#10976=DIRECTION('ref_axis',(1.,0.,0.));
#10977=DIRECTION('center_axis',(0.,0.,1.));
#10978=DIRECTION('ref_axis',(1.,0.,0.));
#10979=DIRECTION('center_axis',(0.,0.,1.));
#10980=DIRECTION('ref_axis',(1.,0.,0.));
#10981=DIRECTION('',(0.,0.,1.));
#10982=DIRECTION('center_axis',(0.,0.,-1.));
#10983=DIRECTION('ref_axis',(1.,0.,0.));
#10984=DIRECTION('center_axis',(0.,0.,1.));
#10985=DIRECTION('ref_axis',(1.,0.,0.));
#10986=DIRECTION('center_axis',(0.,0.,1.));
#10987=DIRECTION('ref_axis',(1.,0.,0.));
#10988=DIRECTION('',(0.,0.,1.));
#10989=DIRECTION('center_axis',(0.,0.,-1.));
#10990=DIRECTION('ref_axis',(1.,0.,0.));
#10991=DIRECTION('center_axis',(0.,0.,1.));
#10992=DIRECTION('ref_axis',(1.,0.,0.));
#10993=DIRECTION('center_axis',(0.,0.,1.));
#10994=DIRECTION('ref_axis',(1.,0.,0.));
#10995=DIRECTION('',(0.,0.,1.));
#10996=DIRECTION('center_axis',(0.,0.,-1.));
#10997=DIRECTION('ref_axis',(1.,0.,0.));
#10998=DIRECTION('center_axis',(0.,0.,1.));
#10999=DIRECTION('ref_axis',(1.,0.,0.));
#11000=DIRECTION('center_axis',(0.,0.,1.));
#11001=DIRECTION('ref_axis',(1.,0.,0.));
#11002=DIRECTION('',(0.,0.,1.));
#11003=DIRECTION('center_axis',(0.,0.,-1.));
#11004=DIRECTION('ref_axis',(1.,0.,0.));
#11005=DIRECTION('center_axis',(0.,0.,1.));
#11006=DIRECTION('ref_axis',(1.,0.,0.));
#11007=DIRECTION('center_axis',(0.,0.,1.));
#11008=DIRECTION('ref_axis',(1.,0.,0.));
#11009=DIRECTION('',(0.,0.,1.));
#11010=DIRECTION('center_axis',(0.,0.,-1.));
#11011=DIRECTION('ref_axis',(1.,0.,0.));
#11012=DIRECTION('center_axis',(0.,0.,1.));
#11013=DIRECTION('ref_axis',(1.,0.,0.));
#11014=DIRECTION('center_axis',(0.,0.,1.));
#11015=DIRECTION('ref_axis',(1.,0.,0.));
#11016=DIRECTION('',(0.,0.,1.));
#11017=DIRECTION('center_axis',(0.,0.,-1.));
#11018=DIRECTION('ref_axis',(1.,0.,0.));
#11019=DIRECTION('center_axis',(0.,0.,1.));
#11020=DIRECTION('ref_axis',(1.,0.,0.));
#11021=DIRECTION('center_axis',(0.,0.,1.));
#11022=DIRECTION('ref_axis',(1.,0.,0.));
#11023=DIRECTION('',(0.,0.,1.));
#11024=DIRECTION('center_axis',(0.,0.,-1.));
#11025=DIRECTION('ref_axis',(1.,0.,0.));
#11026=DIRECTION('center_axis',(0.,0.,1.));
#11027=DIRECTION('ref_axis',(1.,0.,0.));
#11028=DIRECTION('center_axis',(0.,0.,1.));
#11029=DIRECTION('ref_axis',(1.,0.,0.));
#11030=DIRECTION('',(0.,0.,1.));
#11031=DIRECTION('center_axis',(0.,0.,-1.));
#11032=DIRECTION('ref_axis',(1.,0.,0.));
#11033=DIRECTION('center_axis',(0.,0.,1.));
#11034=DIRECTION('ref_axis',(1.,0.,0.));
#11035=DIRECTION('center_axis',(0.,0.,1.));
#11036=DIRECTION('ref_axis',(1.,0.,0.));
#11037=DIRECTION('',(0.,0.,1.));
#11038=DIRECTION('center_axis',(0.,0.,-1.));
#11039=DIRECTION('ref_axis',(1.,0.,0.));
#11040=DIRECTION('center_axis',(0.,0.,1.));
#11041=DIRECTION('ref_axis',(1.,0.,0.));
#11042=DIRECTION('center_axis',(0.,0.,1.));
#11043=DIRECTION('ref_axis',(1.,0.,0.));
#11044=DIRECTION('',(0.,0.,1.));
#11045=DIRECTION('center_axis',(0.,0.,-1.));
#11046=DIRECTION('ref_axis',(1.,0.,0.));
#11047=DIRECTION('center_axis',(0.,0.,1.));
#11048=DIRECTION('ref_axis',(1.,0.,0.));
#11049=DIRECTION('center_axis',(0.,0.,1.));
#11050=DIRECTION('ref_axis',(1.,0.,0.));
#11051=DIRECTION('',(0.,0.,1.));
#11052=DIRECTION('center_axis',(0.,0.,-1.));
#11053=DIRECTION('ref_axis',(1.,0.,0.));
#11054=DIRECTION('center_axis',(0.,0.,1.));
#11055=DIRECTION('ref_axis',(1.,0.,0.));
#11056=DIRECTION('center_axis',(0.,0.,1.));
#11057=DIRECTION('ref_axis',(1.,0.,0.));
#11058=DIRECTION('',(0.,0.,1.));
#11059=DIRECTION('center_axis',(0.,0.,-1.));
#11060=DIRECTION('ref_axis',(1.,0.,0.));
#11061=DIRECTION('center_axis',(0.,0.,1.));
#11062=DIRECTION('ref_axis',(1.,0.,0.));
#11063=DIRECTION('center_axis',(0.,0.,1.));
#11064=DIRECTION('ref_axis',(1.,0.,0.));
#11065=DIRECTION('',(0.,0.,1.));
#11066=DIRECTION('center_axis',(0.,0.,-1.));
#11067=DIRECTION('ref_axis',(1.,0.,0.));
#11068=DIRECTION('center_axis',(0.,0.,1.));
#11069=DIRECTION('ref_axis',(1.,0.,0.));
#11070=DIRECTION('center_axis',(0.,0.,1.));
#11071=DIRECTION('ref_axis',(1.,0.,0.));
#11072=DIRECTION('',(0.,0.,1.));
#11073=DIRECTION('center_axis',(0.,0.,-1.));
#11074=DIRECTION('ref_axis',(1.,0.,0.));
#11075=DIRECTION('center_axis',(0.,0.,1.));
#11076=DIRECTION('ref_axis',(1.,0.,0.));
#11077=DIRECTION('center_axis',(0.,0.,1.));
#11078=DIRECTION('ref_axis',(1.,0.,0.));
#11079=DIRECTION('',(0.,0.,1.));
#11080=DIRECTION('center_axis',(0.,0.,-1.));
#11081=DIRECTION('ref_axis',(1.,0.,0.));
#11082=DIRECTION('center_axis',(0.,0.,1.));
#11083=DIRECTION('ref_axis',(1.,0.,0.));
#11084=DIRECTION('center_axis',(0.,0.,1.));
#11085=DIRECTION('ref_axis',(1.,0.,0.));
#11086=DIRECTION('',(0.,0.,1.));
#11087=DIRECTION('center_axis',(0.,0.,-1.));
#11088=DIRECTION('ref_axis',(1.,0.,0.));
#11089=DIRECTION('center_axis',(0.,0.,1.));
#11090=DIRECTION('ref_axis',(1.,0.,0.));
#11091=DIRECTION('center_axis',(0.,0.,1.));
#11092=DIRECTION('ref_axis',(1.,0.,0.));
#11093=DIRECTION('',(0.,0.,1.));
#11094=DIRECTION('center_axis',(0.,0.,-1.));
#11095=DIRECTION('ref_axis',(1.,0.,0.));
#11096=DIRECTION('center_axis',(0.,0.,1.));
#11097=DIRECTION('ref_axis',(1.,0.,0.));
#11098=DIRECTION('center_axis',(0.,0.,1.));
#11099=DIRECTION('ref_axis',(1.,0.,0.));
#11100=DIRECTION('',(0.,0.,1.));
#11101=DIRECTION('center_axis',(0.,0.,-1.));
#11102=DIRECTION('ref_axis',(1.,0.,0.));
#11103=DIRECTION('center_axis',(0.,0.,1.));
#11104=DIRECTION('ref_axis',(1.,0.,0.));
#11105=DIRECTION('center_axis',(0.,0.,1.));
#11106=DIRECTION('ref_axis',(1.,0.,0.));
#11107=DIRECTION('',(0.,0.,1.));
#11108=DIRECTION('center_axis',(0.,0.,-1.));
#11109=DIRECTION('ref_axis',(1.,0.,0.));
#11110=DIRECTION('center_axis',(0.,1.,0.));
#11111=DIRECTION('ref_axis',(-1.,0.,0.));
#11112=DIRECTION('',(-1.,0.,0.));
#11113=DIRECTION('',(0.,0.,1.));
#11114=DIRECTION('',(-1.,0.,0.));
#11115=DIRECTION('',(0.,0.,1.));
#11116=DIRECTION('center_axis',(1.,0.,0.));
#11117=DIRECTION('ref_axis',(0.,1.,0.));
#11118=DIRECTION('',(0.,1.,0.));
#11119=DIRECTION('',(0.,1.,0.));
#11120=DIRECTION('',(0.,0.,1.));
#11121=DIRECTION('center_axis',(0.,-1.,0.));
#11122=DIRECTION('ref_axis',(1.,0.,0.));
#11123=DIRECTION('',(1.,0.,0.));
#11124=DIRECTION('',(1.,0.,0.));
#11125=DIRECTION('',(0.,0.,1.));
#11126=DIRECTION('center_axis',(-1.,0.,0.));
#11127=DIRECTION('ref_axis',(0.,-1.,0.));
#11128=DIRECTION('',(0.,-1.,0.));
#11129=DIRECTION('',(0.,-1.,0.));
#11130=DIRECTION('center_axis',(0.,0.,1.));
#11131=DIRECTION('ref_axis',(1.,0.,0.));
#11132=DIRECTION('center_axis',(0.,0.,1.));
#11133=DIRECTION('ref_axis',(1.,0.,0.));
#13951=CARTESIAN_POINT('',(0.,0.,0.));
#13952=CARTESIAN_POINT('Origin',(0.,6.,-1.3));
#13953=CARTESIAN_POINT('',(-0.275,6.,-1.2));
#13954=CARTESIAN_POINT('Origin',(0.,6.,-1.2));
#13955=CARTESIAN_POINT('',(-0.275,6.,0.));
#13956=CARTESIAN_POINT('',(-0.275,6.,-1.3));
#13957=CARTESIAN_POINT('Origin',(0.,6.,0.));
#13958=CARTESIAN_POINT('Origin',(0.,-6.,-1.3));
#13959=CARTESIAN_POINT('',(-0.275,-6.,-1.2));
#13960=CARTESIAN_POINT('Origin',(0.,-6.,-1.2));
#13961=CARTESIAN_POINT('',(-0.275,-6.,0.));
#13962=CARTESIAN_POINT('',(-0.275,-6.,-1.3));
#13963=CARTESIAN_POINT('Origin',(0.,-6.,0.));
#13964=CARTESIAN_POINT('Origin',(1.8,-1.8,-1.3));
#13965=CARTESIAN_POINT('',(1.3,-1.8,-1.2));
#13966=CARTESIAN_POINT('Origin',(1.8,-1.8,-1.2));
#13967=CARTESIAN_POINT('',(1.3,-1.8,0.));
#13968=CARTESIAN_POINT('',(1.3,-1.8,-1.3));
#13969=CARTESIAN_POINT('Origin',(1.8,-1.8,0.));
#13970=CARTESIAN_POINT('Origin',(-1.8,1.8,-1.3));
#13971=CARTESIAN_POINT('',(-2.3,1.8,-1.2));
#13972=CARTESIAN_POINT('Origin',(-1.8,1.8,-1.2));
#13973=CARTESIAN_POINT('',(-2.3,1.8,0.));
#13974=CARTESIAN_POINT('',(-2.3,1.8,-1.3));
#13975=CARTESIAN_POINT('Origin',(-1.8,1.8,0.));
#13976=CARTESIAN_POINT('Origin',(-1.8,-1.8,-1.3));
#13977=CARTESIAN_POINT('',(-2.3,-1.8,-1.2));
#13978=CARTESIAN_POINT('Origin',(-1.8,-1.8,-1.2));
#13979=CARTESIAN_POINT('',(-2.3,-1.8,0.));
#13980=CARTESIAN_POINT('',(-2.3,-1.8,-1.3));
#13981=CARTESIAN_POINT('Origin',(-1.8,-1.8,0.));
#13982=CARTESIAN_POINT('Origin',(1.8,1.8,-1.3));
#13983=CARTESIAN_POINT('',(1.3,1.8,-1.2));
#13984=CARTESIAN_POINT('Origin',(1.8,1.8,-1.2));
#13985=CARTESIAN_POINT('',(1.3,1.8,0.));
#13986=CARTESIAN_POINT('',(1.3,1.8,-1.3));
#13987=CARTESIAN_POINT('Origin',(1.8,1.8,0.));
#13988=CARTESIAN_POINT('Origin',(2.9,-2.9,-1.3));
#13989=CARTESIAN_POINT('',(2.69,-2.9,-1.2));
#13990=CARTESIAN_POINT('Origin',(2.9,-2.9,-1.2));
#13991=CARTESIAN_POINT('',(2.69,-2.9,0.));
#13992=CARTESIAN_POINT('',(2.69,-2.9,-1.3));
#13993=CARTESIAN_POINT('Origin',(2.9,-2.9,0.));
#13994=CARTESIAN_POINT('Origin',(-2.9,2.9,-1.3));
#13995=CARTESIAN_POINT('',(-3.11,2.9,-1.2));
#13996=CARTESIAN_POINT('Origin',(-2.9,2.9,-1.2));
#13997=CARTESIAN_POINT('',(-3.11,2.9,0.));
#13998=CARTESIAN_POINT('',(-3.11,2.9,-1.3));
#13999=CARTESIAN_POINT('Origin',(-2.9,2.9,0.));
#14000=CARTESIAN_POINT('Origin',(-2.9,-2.9,-1.3));
#14001=CARTESIAN_POINT('',(-3.11,-2.9,-1.2));
#14002=CARTESIAN_POINT('Origin',(-2.9,-2.9,-1.2));
#14003=CARTESIAN_POINT('',(-3.11,-2.9,0.));
#14004=CARTESIAN_POINT('',(-3.11,-2.9,-1.3));
#14005=CARTESIAN_POINT('Origin',(-2.9,-2.9,0.));
#14006=CARTESIAN_POINT('Origin',(2.9,2.9,-1.3));
#14007=CARTESIAN_POINT('',(2.69,2.9,-1.2));
#14008=CARTESIAN_POINT('Origin',(2.9,2.9,-1.2));
#14009=CARTESIAN_POINT('',(2.69,2.9,0.));
#14010=CARTESIAN_POINT('',(2.69,2.9,-1.3));
#14011=CARTESIAN_POINT('Origin',(2.9,2.9,0.));
#14012=CARTESIAN_POINT('Origin',(4.4,6.7,-1.3));
#14013=CARTESIAN_POINT('',(4.125,6.7,-1.2));
#14014=CARTESIAN_POINT('Origin',(4.4,6.7,-1.2));
#14015=CARTESIAN_POINT('',(4.125,6.7,0.));
#14016=CARTESIAN_POINT('',(4.125,6.7,-1.3));
#14017=CARTESIAN_POINT('Origin',(4.4,6.7,0.));
#14018=CARTESIAN_POINT('Origin',(7.6,6.7,-1.3));
#14019=CARTESIAN_POINT('',(7.325,6.7,-1.2));
#14020=CARTESIAN_POINT('Origin',(7.6,6.7,-1.2));
#14021=CARTESIAN_POINT('',(7.325,6.7,0.));
#14022=CARTESIAN_POINT('',(7.325,6.7,-1.3));
#14023=CARTESIAN_POINT('Origin',(7.6,6.7,0.));
#14024=CARTESIAN_POINT('Origin',(4.4,-1.3,-1.3));
#14025=CARTESIAN_POINT('',(4.125,-1.3,-1.2));
#14026=CARTESIAN_POINT('Origin',(4.4,-1.3,-1.2));
#14027=CARTESIAN_POINT('',(4.125,-1.3,0.));
#14028=CARTESIAN_POINT('',(4.125,-1.3,-1.3));
#14029=CARTESIAN_POINT('Origin',(4.4,-1.3,0.));
#14030=CARTESIAN_POINT('Origin',(7.6,-1.3,-1.3));
#14031=CARTESIAN_POINT('',(7.325,-1.3,-1.2));
#14032=CARTESIAN_POINT('Origin',(7.6,-1.3,-1.2));
#14033=CARTESIAN_POINT('',(7.325,-1.3,0.));
#14034=CARTESIAN_POINT('',(7.325,-1.3,-1.3));
#14035=CARTESIAN_POINT('Origin',(7.6,-1.3,0.));
#14036=CARTESIAN_POINT('Origin',(-7.6,6.7,-1.3));
#14037=CARTESIAN_POINT('',(-7.875,6.7,-1.2));
#14038=CARTESIAN_POINT('Origin',(-7.6,6.7,-1.2));
#14039=CARTESIAN_POINT('',(-7.875,6.7,0.));
#14040=CARTESIAN_POINT('',(-7.875,6.7,-1.3));
#14041=CARTESIAN_POINT('Origin',(-7.6,6.7,0.));
#14042=CARTESIAN_POINT('Origin',(-4.4,6.7,-1.3));
#14043=CARTESIAN_POINT('',(-4.675,6.7,-1.2));
#14044=CARTESIAN_POINT('Origin',(-4.4,6.7,-1.2));
#14045=CARTESIAN_POINT('',(-4.675,6.7,0.));
#14046=CARTESIAN_POINT('',(-4.675,6.7,-1.3));
#14047=CARTESIAN_POINT('Origin',(-4.4,6.7,0.));
#14048=CARTESIAN_POINT('Origin',(-7.6,-1.3,-1.3));
#14049=CARTESIAN_POINT('',(-7.875,-1.3,-1.2));
#14050=CARTESIAN_POINT('Origin',(-7.6,-1.3,-1.2));
#14051=CARTESIAN_POINT('',(-7.875,-1.3,0.));
#14052=CARTESIAN_POINT('',(-7.875,-1.3,-1.3));
#14053=CARTESIAN_POINT('Origin',(-7.6,-1.3,0.));
#14054=CARTESIAN_POINT('Origin',(-4.4,-1.3,-1.3));
#14055=CARTESIAN_POINT('',(-4.675,-1.3,-1.2));
#14056=CARTESIAN_POINT('Origin',(-4.4,-1.3,-1.2));
#14057=CARTESIAN_POINT('',(-4.675,-1.3,0.));
#14058=CARTESIAN_POINT('',(-4.675,-1.3,-1.3));
#14059=CARTESIAN_POINT('Origin',(-4.4,-1.3,0.));
#14060=CARTESIAN_POINT('Origin',(9.5,10.,-1.3));
#14061=CARTESIAN_POINT('',(9.225,10.,-1.2));
#14062=CARTESIAN_POINT('Origin',(9.5,10.,-1.2));
#14063=CARTESIAN_POINT('',(9.225,10.,0.));
#14064=CARTESIAN_POINT('',(9.225,10.,-1.3));
#14065=CARTESIAN_POINT('Origin',(9.5,10.,0.));
#14066=CARTESIAN_POINT('Origin',(9.5,11.,-1.3));
#14067=CARTESIAN_POINT('',(9.225,11.,-1.2));
#14068=CARTESIAN_POINT('Origin',(9.5,11.,-1.2));
#14069=CARTESIAN_POINT('',(9.225,11.,0.));
#14070=CARTESIAN_POINT('',(9.225,11.,-1.3));
#14071=CARTESIAN_POINT('Origin',(9.5,11.,0.));
#14072=CARTESIAN_POINT('Origin',(-9.5,10.,-1.3));
#14073=CARTESIAN_POINT('',(-9.775,10.,-1.2));
#14074=CARTESIAN_POINT('Origin',(-9.5,10.,-1.2));
#14075=CARTESIAN_POINT('',(-9.775,10.,0.));
#14076=CARTESIAN_POINT('',(-9.775,10.,-1.3));
#14077=CARTESIAN_POINT('Origin',(-9.5,10.,0.));
#14078=CARTESIAN_POINT('Origin',(-9.5,11.,-1.3));
#14079=CARTESIAN_POINT('',(-9.775,11.,-1.2));
#14080=CARTESIAN_POINT('Origin',(-9.5,11.,-1.2));
#14081=CARTESIAN_POINT('',(-9.775,11.,0.));
#14082=CARTESIAN_POINT('',(-9.775,11.,-1.3));
#14083=CARTESIAN_POINT('Origin',(-9.5,11.,0.));
#14084=CARTESIAN_POINT('Origin',(11.,12.5,-1.2));
#14085=CARTESIAN_POINT('',(11.,12.5,-1.2));
#14086=CARTESIAN_POINT('',(-11.,12.5,-1.2));
#14087=CARTESIAN_POINT('',(11.,12.5,-1.2));
#14088=CARTESIAN_POINT('',(-11.,12.5,0.));
#14089=CARTESIAN_POINT('',(-11.,12.5,-1.2));
#14090=CARTESIAN_POINT('',(11.,12.5,0.));
#14091=CARTESIAN_POINT('',(11.,12.5,0.));
#14092=CARTESIAN_POINT('',(11.,12.5,-1.2));
#14093=CARTESIAN_POINT('Origin',(11.,-8.,-1.2));
#14094=CARTESIAN_POINT('',(11.,-8.,-1.2));
#14095=CARTESIAN_POINT('',(11.,-8.,-1.2));
#14096=CARTESIAN_POINT('',(11.,-8.,0.));
#14097=CARTESIAN_POINT('',(11.,-8.,0.));
#14098=CARTESIAN_POINT('',(11.,-8.,-1.2));
#14099=CARTESIAN_POINT('Origin',(-11.,-8.,-1.2));
#14100=CARTESIAN_POINT('',(-11.,-8.,-1.2));
#14101=CARTESIAN_POINT('',(-11.,-8.,-1.2));
#14102=CARTESIAN_POINT('',(-11.,-8.,0.));
#14103=CARTESIAN_POINT('',(-11.,-8.,0.));
#14104=CARTESIAN_POINT('',(-11.,-8.,-1.2));
#14105=CARTESIAN_POINT('Origin',(-11.,12.5,-1.2));
#14106=CARTESIAN_POINT('',(-11.,12.5,-1.2));
#14107=CARTESIAN_POINT('',(-11.,12.5,0.));
#14108=CARTESIAN_POINT('Origin',(0.,2.25,0.));
#14109=CARTESIAN_POINT('Origin',(0.,2.25,-1.2));
#22295=UNCERTAINTY_MEASURE_WITH_UNIT(LENGTH_MEASURE(0.001),#22395,
'DISTANCE_ACCURACY_VALUE',
'Maximum model space distance between geometric entities at asserted c
onnectivities');
#22343=UNCERTAINTY_MEASURE_WITH_UNIT(LENGTH_MEASURE(0.001),#22395,
'DISTANCE_ACCURACY_VALUE',
'Maximum model space distance between geometric entities at asserted c
onnectivities');
#22346=(
GEOMETRIC_REPRESENTATION_CONTEXT(3)
GLOBAL_UNCERTAINTY_ASSIGNED_CONTEXT((#22295))
GLOBAL_UNIT_ASSIGNED_CONTEXT((#22395,#22397,#22398))
REPRESENTATION_CONTEXT('','3D')
);
#22394=(
GEOMETRIC_REPRESENTATION_CONTEXT(3)
GLOBAL_UNCERTAINTY_ASSIGNED_CONTEXT((#22343))
GLOBAL_UNIT_ASSIGNED_CONTEXT((#22395,#22397,#22398))
REPRESENTATION_CONTEXT('','3D')
);
#22395=(
LENGTH_UNIT()
NAMED_UNIT(*)
SI_UNIT(.CENTI.,.METRE.)
);
#22397=(
NAMED_UNIT(*)
PLANE_ANGLE_UNIT()
SI_UNIT($,.RADIAN.)
);
#22398=(
NAMED_UNIT(*)
SI_UNIT($,.STERADIAN.)
SOLID_ANGLE_UNIT()
);
#22401=SHAPE_DEFINITION_REPRESENTATION(#22451,#22640);
#22451=PRODUCT_DEFINITION_SHAPE('',$,#22691);
#22640=SHAPE_REPRESENTATION('',(#9762),#22346);
#22688=PRODUCT_DEFINITION_CONTEXT('part definition',#22840,'design');
#22691=PRODUCT_DEFINITION('Base','Base',#22741,#22688);
#22741=PRODUCT_DEFINITION_FORMATION('',$,#22844);
#22840=APPLICATION_CONTEXT(
'Core Data for Automotive Mechanical Design Process');
#22841=PRODUCT_CONTEXT('part definition',#22840,'mechanical');
#22844=PRODUCT('Base','Base','Base',(#22841));
#22934=COLOUR_RGB('Dark Blue',0.08,0.2,0.34);
#22935=FILL_AREA_STYLE_COLOUR('',#22934);
#22936=FILL_AREA_STYLE('',(#22935));
#22937=SURFACE_STYLE_FILL_AREA(#22936);
#22938=SURFACE_SIDE_STYLE('',(#22937));
#22939=SURFACE_STYLE_USAGE(.BOTH.,#22938);
#22940=PRESENTATION_STYLE_ASSIGNMENT((#22939));
ENDSEC;
END-ISO-10303-21;
